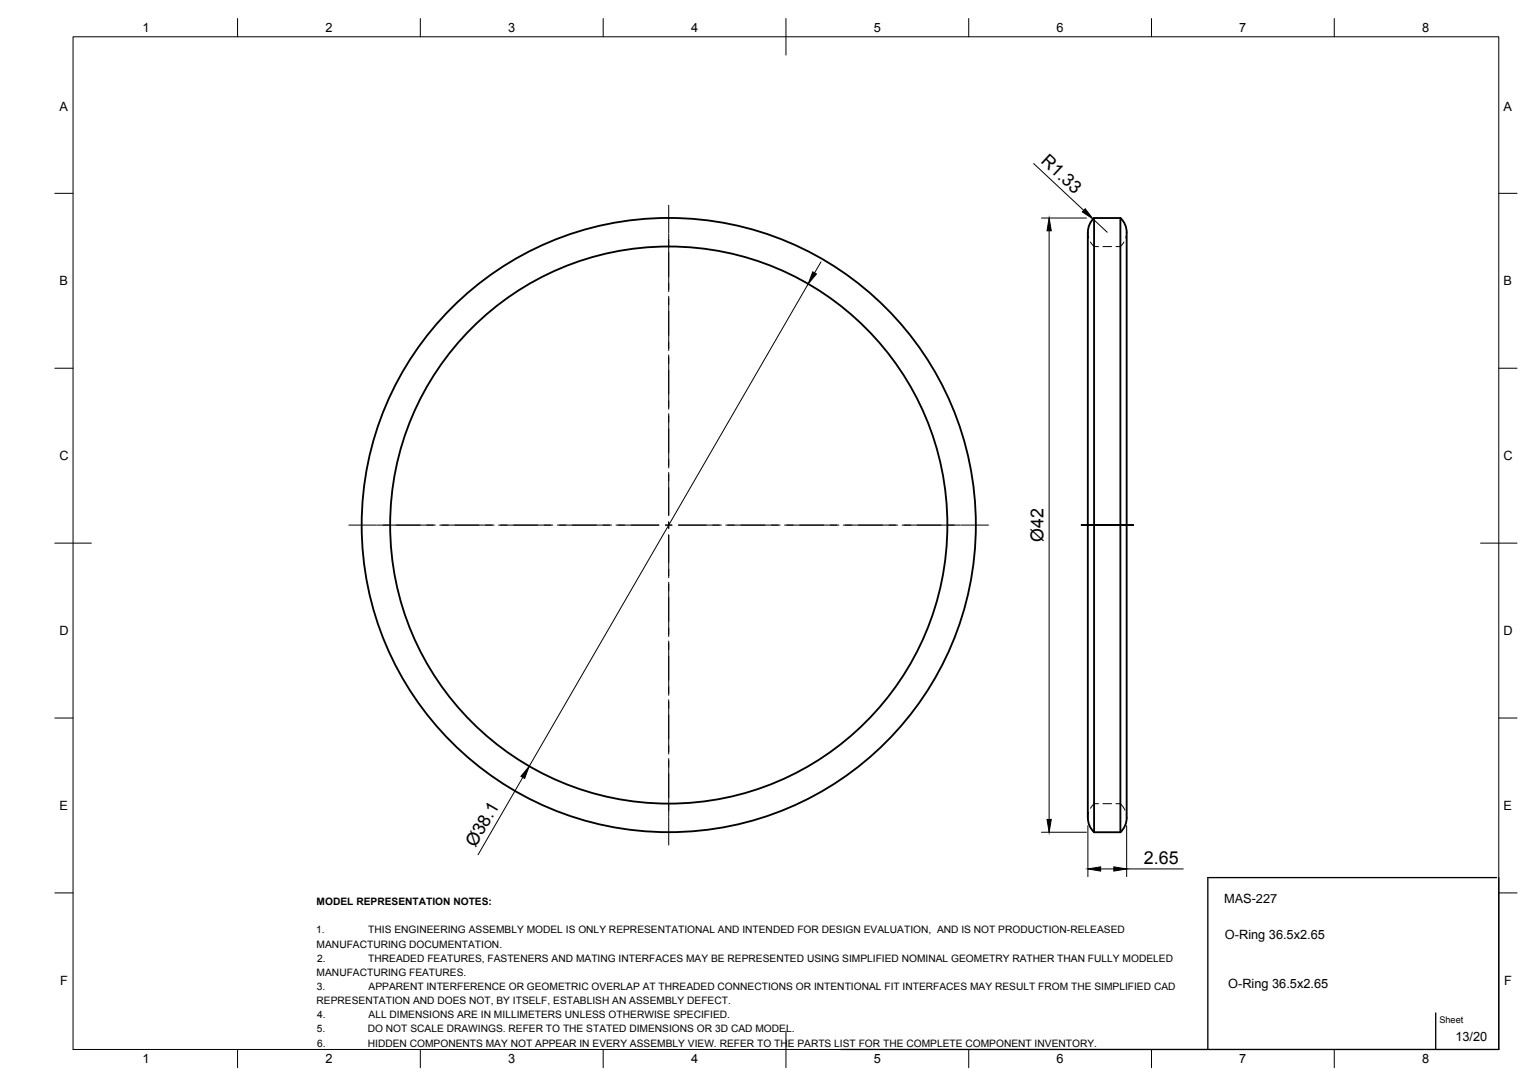
ISO-10303-21;
HEADER;
FILE_DESCRIPTION (('STEP AP214'),
    '1' );
FILE_NAME ( 'O-Ring 36.5x2.65.step', '2026-10-06T08:24:41', ( '' ), ( '' ), 'STEP AP214', 'Unspecified', '' );
FILE_SCHEMA (( 'AUTOMOTIVE_DESIGN' ));
ENDSEC;
DATA;
#54=DIRECTION ( 'NONE',  ( 1.000000000000000000, 0.000000000000000000, 0.000000000000000000 ) ) ;
#154=ADVANCED_FACE ( 'NONE', ( #2979 ), #26440, .T. ) ;
#275=ORIENTED_EDGE ( 'NONE', *, *, #12081, .F. ) ;
#358=DIRECTION ( 'NONE',  ( 0.000000000000000000, 0.000000000000000000, -1.000000000000000000 ) ) ;
#727=AXIS2_PLACEMENT_3D ( 'NONE', #14437, #3821, #3372 ) ;
#893=DIRECTION ( 'NONE',  ( 0.000000000000000000, 1.000000000000000000, 0.000000000000000000 ) ) ;
#953=DIRECTION ( 'NONE',  ( 1.000000000000000000, 0.000000000000000000, 0.000000000000000000 ) ) ;
#1494=CARTESIAN_POINT ( 'NONE',  ( -0.03532354024591893848, -0.07677165354330710290, 0.000000000000000000 ) ) ;
#1499=ORIENTED_EDGE ( 'NONE', *, *, #6385, .T. ) ;
#1533=PRODUCT_DEFINITION ( 'UNKNOWN', '', #2104, #3431 ) ;
#1669=ORIENTED_EDGE ( 'NONE', *, *, #3115, .T. ) ;
#1764=DIRECTION ( 'NONE',  ( 0.000000000000000000, 1.000000000000000000, 0.000000000000000000 ) ) ;
#1788=EDGE_CURVE ( 'NONE', #6256, #18898, #12424, .T. ) ;
#1859=ORIENTED_EDGE ( 'NONE', *, *, #22214, .F. ) ;
#1926=DIRECTION ( 'NONE',  ( 1.000000000000000000, 0.000000000000000000, 0.000000000000000000 ) ) ;
#2043=EDGE_CURVE ( 'NONE', #17434, #11924, #21465, .T. ) ;
#2104=PRODUCT_DEFINITION_FORMATION_WITH_SPECIFIED_SOURCE ( 'ANY', '', #22884, .NOT_KNOWN. ) ;
#2296=CARTESIAN_POINT ( 'NONE',  ( -9.069736220472442904E-16, -0.8267716535433071723, 0.000000000000000000 ) ) ;
#2375=EDGE_LOOP ( 'NONE', ( #25682, #7320, #24025, #12399, #13275, #4753 ) ) ;
#2557=ORIENTED_EDGE ( 'NONE', *, *, #12567, .F. ) ;
#2568=FACE_OUTER_BOUND ( 'NONE', #25010, .T. ) ;
#2659=ORIENTED_EDGE ( 'NONE', *, *, #23278, .F. ) ;
#2715=AXIS2_PLACEMENT_3D ( 'NONE', #11396, #22136, #24804 ) ;
#2813=AXIS2_PLACEMENT_3D ( 'NONE', #9732, #3355, #3801 ) ;
#2979=FACE_OUTER_BOUND ( 'NONE', #26175, .T. ) ;
#3059=( CONVERSION_BASED_UNIT ( 'INCH', #5779 ) LENGTH_UNIT ( ) NAMED_UNIT ( #6927 ) ) ;
#3098=EDGE_CURVE ( 'NONE', #18478, #18898, #7298, .T. ) ;
#3105=APPLICATION_CONTEXT ( 'automotive_design' ) ;
#3115=EDGE_CURVE ( 'NONE', #27881, #10521, #9696, .T. ) ;
#3269=DIRECTION ( 'NONE',  ( 0.000000000000000000, 1.000000000000000000, 0.000000000000000000 ) ) ;
#3355=DIRECTION ( 'NONE',  ( 1.000000000000000000, 0.000000000000000000, 0.000000000000000000 ) ) ;
#3372=DIRECTION ( 'NONE',  ( 1.000000000000000000, 0.000000000000000000, 0.000000000000000000 ) ) ;
#3431=PRODUCT_DEFINITION_CONTEXT ( 'detailed design', #3105, 'design' ) ;
#3439=DIRECTION ( 'NONE',  ( 1.000000000000000000, 0.000000000000000000, 0.000000000000000000 ) ) ;
#3497=VECTOR ( 'NONE', #20294, 39.37007874015748143 ) ;
#3512=AXIS2_PLACEMENT_3D ( 'NONE', #10785, #15718, #19545 ) ;
#3517=ORIENTED_EDGE ( 'NONE', *, *, #3621, .T. ) ;
#3592=ADVANCED_FACE ( 'NONE', ( #2568 ), #20689, .T. ) ;
#3621=EDGE_CURVE ( 'NONE', #16090, #10521, #23858, .T. ) ;
#3665=DIRECTION ( 'NONE',  ( 0.000000000000000000, 0.000000000000000000, 1.000000000000000000 ) ) ;
#3718=ORIENTED_EDGE ( 'NONE', *, *, #6749, .F. ) ;
#3738=CIRCLE ( 'NONE', #17721, 0.7500000000000001110 ) ;
#3801=DIRECTION ( 'NONE',  ( 0.000000000000000000, 1.000000000000000000, 0.000000000000000000 ) ) ;
#3821=DIRECTION ( 'NONE',  ( -1.147443000000000016E-15, -1.000000000000000000, -0.000000000000000000 ) ) ;
#4013=DIRECTION ( 'NONE',  ( 1.147443000000000016E-15, 1.000000000000000000, -1.224646799147353207E-16 ) ) ;
#4081=ORIENTED_EDGE ( 'NONE', *, *, #2043, .T. ) ;
#4143=COLOUR_RGB ( '', 0.31764706, 0.68627451, 0.89019608) ;
#4379=CIRCLE ( 'NONE', #4458, 0.7500000000000001110 ) ;
#4413=AXIS2_PLACEMENT_3D ( 'NONE', #15060, #6843, #7242 ) ;
#4458=AXIS2_PLACEMENT_3D ( 'NONE', #13653, #953, #22137 ) ;
#4753=ORIENTED_EDGE ( 'NONE', *, *, #15365, .F. ) ;
#5004=AXIS2_PLACEMENT_3D ( 'NONE', #6179, #23951, #19289 ) ;
#5229=CARTESIAN_POINT ( 'NONE',  ( 0.000000000000000000, 0.000000000000000000, 0.000000000000000000 ) ) ;
#5350=CIRCLE ( 'NONE', #9865, 0.8267716535433071723 ) ;
#5380=CIRCLE ( 'NONE', #23912, 0.7500000000000001110 ) ;
#5383=CARTESIAN_POINT ( 'NONE',  ( -9.069736220472440932E-16, -0.8267716535433070613, 0.7883858267716535861 ) ) ;
#5415=SHAPE_REPRESENTATION ( 'O-Ring 36.5x2.65', ( #11588 ), #12073 ) ;
#5431=CARTESIAN_POINT ( 'NONE',  ( -0.03532354024591901481, -0.8267716535433070613, 0.8267716535433070613 ) ) ;
#5548=TOROIDAL_SURFACE ( 'NONE', #20874, 0.7883858267716535861, 0.05216535433070866590 ) ;
#5658=AXIS2_PLACEMENT_3D ( 'NONE', #16841, #14751, #17254 ) ;
#5779=LENGTH_MEASURE_WITH_UNIT ( LENGTH_MEASURE( 0.02539999999999999897 ), #11694 ) ;
#5900=CARTESIAN_POINT ( 'NONE',  ( 0.03532354024591720376, -0.07677165354330710290, 0.000000000000000000 ) ) ;
#5969=DIRECTION ( 'NONE',  ( 1.000000000000000000, 0.000000000000000000, 0.000000000000000000 ) ) ;
#6179=CARTESIAN_POINT ( 'NONE',  ( 0.03532354024591720376, -0.8267716535433071723, 0.000000000000000000 ) ) ;
#6256=VERTEX_POINT ( 'NONE', #16209 ) ;
#6276=VERTEX_POINT ( 'NONE', #5900 ) ;
#6323=VECTOR ( 'NONE', #1926, 39.37007874015748143 ) ;
#6347=AXIS2_PLACEMENT_3D ( 'NONE', #26823, #11849, #7473 ) ;
#6385=EDGE_CURVE ( 'NONE', #17999, #18223, #25936, .T. ) ;
#6400=EDGE_LOOP ( 'NONE', ( #14006, #9282, #3718, #18640, #19761, #26637 ) ) ;
#6472=EDGE_LOOP ( 'NONE', ( #24744, #21279, #20965, #19101, #24711, #8476 ) ) ;
#6507=ORIENTED_EDGE ( 'NONE', *, *, #8834, .F. ) ;
#6607=CIRCLE ( 'NONE', #727, 0.05216535433070866590 ) ;
#6629=ADVANCED_FACE ( 'NONE', ( #27518 ), #24064, .F. ) ;
#6697=DIRECTION ( 'NONE',  ( 1.000000000000000000, 0.000000000000000000, 0.000000000000000000 ) ) ;
#6749=EDGE_CURVE ( 'NONE', #11924, #14095, #11728, .T. ) ;
#6843=DIRECTION ( 'NONE',  ( 1.000000000000000000, 0.000000000000000000, 0.000000000000000000 ) ) ;
#6927=DIMENSIONAL_EXPONENTS ( 1.000000000000000000, 0.000000000000000000, 0.000000000000000000, 0.000000000000000000, 0.000000000000000000, 0.000000000000000000, 0.000000000000000000 ) ;
#6933=SURFACE_SIDE_STYLE ('',( #26000 ) ) ;
#7013=AXIS2_PLACEMENT_3D ( 'NONE', #26658, #20166, #26383 ) ;
#7106=CARTESIAN_POINT ( 'NONE',  ( -9.506830708661417994E-16, -0.8267716535433071723, 0.000000000000000000 ) ) ;
#7112=CARTESIAN_POINT ( 'NONE',  ( 0.03532354024591712049, -0.8267716535433071723, 0.000000000000000000 ) ) ;
#7199=CIRCLE ( 'NONE', #9438, 0.7500000000000001110 ) ;
#7242=DIRECTION ( 'NONE',  ( 0.000000000000000000, 1.000000000000000000, 0.000000000000000000 ) ) ;
#7259=ADVANCED_FACE ( 'NONE', ( #13509 ), #7434, .F. ) ;
#7265=CARTESIAN_POINT ( 'NONE',  ( -9.069736220472442904E-16, -0.8267716535433071723, 0.000000000000000000 ) ) ;
#7298=LINE ( 'NONE', #9261, #3497 ) ;
#7320=ORIENTED_EDGE ( 'NONE', *, *, #18108, .T. ) ;
#7427=DIRECTION ( 'NONE',  ( 0.000000000000000000, 1.000000000000000000, 0.000000000000000000 ) ) ;
#7434=CYLINDRICAL_SURFACE ( 'NONE', #2715, 0.7500000000000001110 ) ;
#7473=DIRECTION ( 'NONE',  ( 0.000000000000000000, 1.000000000000000000, 0.000000000000000000 ) ) ;
#7497=AXIS2_PLACEMENT_3D ( 'NONE', #22749, #18351, #12293 ) ;
#7529=DIRECTION ( 'NONE',  ( 1.000000000000000000, 0.000000000000000000, 0.000000000000000000 ) ) ;
#7625=CYLINDRICAL_SURFACE ( 'NONE', #2813, 0.8267716535433071723 ) ;
#7667=ORIENTED_EDGE ( 'NONE', *, *, #20733, .T. ) ;
#7694=ORIENTED_EDGE ( 'NONE', *, *, #23278, .T. ) ;
#7752=EDGE_LOOP ( 'NONE', ( #7667, #22292, #1669, #20527, #1859, #13973 ) ) ;
#7757=EDGE_CURVE ( 'NONE', #23920, #6276, #9061, .T. ) ;
#7770=PRODUCT_DEFINITION_SHAPE ( 'NONE', 'NONE',  #1533 ) ;
#7923=DIRECTION ( 'NONE',  ( 1.000000000000000000, 0.000000000000000000, 0.000000000000000000 ) ) ;
#7957=VERTEX_POINT ( 'NONE', #5431 ) ;
#7970=ORIENTED_EDGE ( 'NONE', *, *, #2043, .F. ) ;
#8012=CARTESIAN_POINT ( 'NONE',  ( 0.03532354024591720376, -1.576771653543307172, 9.184850993605150903E-17 ) ) ;
#8080=CARTESIAN_POINT ( 'NONE',  ( -0.03532354024591893848, -0.8267716535433071723, -0.7500000000000001110 ) ) ;
#8084=CARTESIAN_POINT ( 'NONE',  ( 0.03532354024591712049, -0.8267716535433071723, 0.000000000000000000 ) ) ;
#8218=DIRECTION ( 'NONE',  ( 1.000000000000000000, 0.000000000000000000, 0.000000000000000000 ) ) ;
#8410=DIRECTION ( 'NONE',  ( 1.000000000000000000, 0.000000000000000000, 0.000000000000000000 ) ) ;
#8476=ORIENTED_EDGE ( 'NONE', *, *, #1788, .T. ) ;
#8487=( CONVERSION_BASED_UNIT ( 'INCH', #10883 ) LENGTH_UNIT ( ) NAMED_UNIT ( #22953 ) ) ;
#8506=EDGE_CURVE ( 'NONE', #14095, #7957, #15004, .T. ) ;
#8613=DIRECTION ( 'NONE',  ( 1.000000000000000000, 0.000000000000000000, 0.000000000000000000 ) ) ;
#8620=DIRECTION ( 'NONE',  ( 0.000000000000000000, 1.000000000000000000, 0.000000000000000000 ) ) ;
#8834=EDGE_CURVE ( 'NONE', #11924, #6276, #27573, .T. ) ;
#8969=FACE_OUTER_BOUND ( 'NONE', #16226, .T. ) ;
#9030=FILL_AREA_STYLE_COLOUR ( '', #4143 ) ;
#9061=CIRCLE ( 'NONE', #5004, 0.7500000000000001110 ) ;
#9258=ADVANCED_FACE ( 'NONE', ( #16380 ), #7625, .T. ) ;
#9261=CARTESIAN_POINT ( 'NONE',  ( -9.506830708661417994E-16, 0.000000000000000000, 0.000000000000000000 ) ) ;
#9282=ORIENTED_EDGE ( 'NONE', *, *, #18108, .F. ) ;
#9337=DIRECTION ( 'NONE',  ( 1.000000000000000000, 0.000000000000000000, 0.000000000000000000 ) ) ;
#9392=DIRECTION ( 'NONE',  ( 1.000000000000000000, 0.000000000000000000, 0.000000000000000000 ) ) ;
#9438=AXIS2_PLACEMENT_3D ( 'NONE', #21199, #8613, #27031 ) ;
#9531=VECTOR ( 'NONE', #8218, 39.37007874015748143 ) ;
#9601=DIRECTION ( 'NONE',  ( 1.147443000000000016E-15, 1.000000000000000000, -1.224646799147353207E-16 ) ) ;
#9630=DIRECTION ( 'NONE',  ( 0.000000000000000000, 1.000000000000000000, 0.000000000000000000 ) ) ;
#9696=LINE ( 'NONE', #18296, #11621 ) ;
#9732=CARTESIAN_POINT ( 'NONE',  ( -9.506830708661417994E-16, -0.8267716535433071723, 0.000000000000000000 ) ) ;
#9750=CARTESIAN_POINT ( 'NONE',  ( -0.03532354024591901481, -1.653543307086614345, 1.012503259137575512E-16 ) ) ;
#9859=( NAMED_UNIT ( * ) SI_UNIT ( $, .STERADIAN. ) SOLID_ANGLE_UNIT ( ) ) ;
#9865=AXIS2_PLACEMENT_3D ( 'NONE', #19355, #54, #8620 ) ;
#10041=CARTESIAN_POINT ( 'NONE',  ( -8.632637795275590524E-16, -0.07677165354330710290, 0.000000000000000000 ) ) ;
#10188=CIRCLE ( 'NONE', #21950, 0.05216535433070866590 ) ;
#10458=AXIS2_PLACEMENT_3D ( 'NONE', #27460, #4013, #20958 ) ;
#10521=VERTEX_POINT ( 'NONE', #17065 ) ;
#10785=CARTESIAN_POINT ( 'NONE',  ( 0.03532354024591712049, -0.8267716535433071723, 0.000000000000000000 ) ) ;
#10857=AXIS2_PLACEMENT_3D ( 'NONE', #15408, #16853, #18661 ) ;
#10883=LENGTH_MEASURE_WITH_UNIT ( LENGTH_MEASURE( 0.02539999999999999897 ), #19498 ) ;
#11131=ORIENTED_EDGE ( 'NONE', *, *, #11690, .F. ) ;
#11208=AXIS2_PLACEMENT_3D ( 'NONE', #8084, #5969, #18942 ) ;
#11396=CARTESIAN_POINT ( 'NONE',  ( -8.632637795275590524E-16, -0.8267716535433071723, 0.000000000000000000 ) ) ;
#11588=AXIS2_PLACEMENT_3D ( 'NONE', #5229, #3665, #7923 ) ;
#11621=VECTOR ( 'NONE', #22138, 39.37007874015748143 ) ;
#11690=EDGE_CURVE ( 'NONE', #18223, #23920, #3738, .T. ) ;
#11694=( LENGTH_UNIT ( ) NAMED_UNIT ( * ) SI_UNIT ( $, .METRE. ) ) ;
#11728=CIRCLE ( 'NONE', #6347, 0.7500000000000001110 ) ;
#11849=DIRECTION ( 'NONE',  ( 1.000000000000000000, 0.000000000000000000, 0.000000000000000000 ) ) ;
#11924=VERTEX_POINT ( 'NONE', #1494 ) ;
#11936=CIRCLE ( 'NONE', #18673, 0.8267716535433071723 ) ;
#11990=VERTEX_POINT ( 'NONE', #22499 ) ;
#12073=( GEOMETRIC_REPRESENTATION_CONTEXT ( 3 ) GLOBAL_UNCERTAINTY_ASSIGNED_CONTEXT ( ( #18691 ) ) GLOBAL_UNIT_ASSIGNED_CONTEXT ( ( #3059, #16228, #9859 ) ) REPRESENTATION_CONTEXT ( 'NONE', 'WORKASPACE' ) ) ;
#12081=EDGE_CURVE ( 'NONE', #17434, #14806, #21229, .T. ) ;
#12293=DIRECTION ( 'NONE',  ( 0.000000000000000000, 0.000000000000000000, -1.000000000000000000 ) ) ;
#12381=CARTESIAN_POINT ( 'NONE',  ( -8.632637795275590524E-16, -1.576771653543307172, 9.184850993605150903E-17 ) ) ;
#12399=ORIENTED_EDGE ( 'NONE', *, *, #12081, .T. ) ;
#12424=CIRCLE ( 'NONE', #19193, 0.8267716535433071723 ) ;
#12567=EDGE_CURVE ( 'NONE', #11990, #18223, #21732, .T. ) ;
#12719=FILL_AREA_STYLE ('',( #9030 ) ) ;
#12811=ORIENTED_EDGE ( 'NONE', *, *, #22158, .T. ) ;
#13232=ORIENTED_EDGE ( 'NONE', *, *, #6749, .T. ) ;
#13259=ADVANCED_FACE ( 'NONE', ( #8969 ), #5548, .T. ) ;
#13275=ORIENTED_EDGE ( 'NONE', *, *, #19557, .F. ) ;
#13364=ORIENTED_EDGE ( 'NONE', *, *, #22350, .F. ) ;
#13390=DIRECTION ( 'NONE',  ( 0.000000000000000000, 1.000000000000000000, 0.000000000000000000 ) ) ;
#13444=DIRECTION ( 'NONE',  ( 1.000000000000000000, -1.147443000000000016E-15, 0.000000000000000000 ) ) ;
#13509=FACE_OUTER_BOUND ( 'NONE', #6400, .T. ) ;
#13515=CARTESIAN_POINT ( 'NONE',  ( 0.03532354024591720376, -0.8267716535433071723, -0.7500000000000001110 ) ) ;
#13653=CARTESIAN_POINT ( 'NONE',  ( -0.03532354024591893848, -0.8267716535433071723, 0.000000000000000000 ) ) ;
#13973=ORIENTED_EDGE ( 'NONE', *, *, #3098, .F. ) ;
#14006=ORIENTED_EDGE ( 'NONE', *, *, #6385, .F. ) ;
#14057=STYLED_ITEM ( 'NONE', ( #21627 ), #21602 ) ;
#14095=VERTEX_POINT ( 'NONE', #17627 ) ;
#14303=ORIENTED_EDGE ( 'NONE', *, *, #3098, .T. ) ;
#14351=CARTESIAN_POINT ( 'NONE',  ( 0.03532354024591720376, -0.8267716535433071723, 0.000000000000000000 ) ) ;
#14437=CARTESIAN_POINT ( 'NONE',  ( -9.069736220472442904E-16, -0.8267716535433071723, -0.7883858267716535861 ) ) ;
#14453=ORIENTED_EDGE ( 'NONE', *, *, #7757, .T. ) ;
#14655=CARTESIAN_POINT ( 'NONE',  ( -0.03532354024591901481, -0.8267716535433071723, 0.000000000000000000 ) ) ;
#14695=SHAPE_REPRESENTATION_RELATIONSHIP ( 'NONE' , 'NONE' ,  #5415, #17421 ) ;
#14751=DIRECTION ( 'NONE',  ( 1.000000000000000000, -1.147443000000000016E-15, 0.000000000000000000 ) ) ;
#14806=VERTEX_POINT ( 'NONE', #15024 ) ;
#14979=CARTESIAN_POINT ( 'NONE',  ( -0.03532354024591893848, -1.576771653543307172, 9.184850993605150903E-17 ) ) ;
#15004=CIRCLE ( 'NONE', #10458, 0.05216535433070866590 ) ;
#15024=CARTESIAN_POINT ( 'NONE',  ( -0.03532354024591901481, -0.8267716535433071723, -0.8267716535433070613 ) ) ;
#15060=CARTESIAN_POINT ( 'NONE',  ( -0.03532354024591901481, -0.8267716535433071723, 0.000000000000000000 ) ) ;
#15184=TOROIDAL_SURFACE ( 'NONE', #7497, 0.7883858267716535861, 0.05216535433070866590 ) ;
#15256=AXIS2_PLACEMENT_3D ( 'NONE', #7112, #7529, #3269 ) ;
#15365=EDGE_CURVE ( 'NONE', #7957, #27881, #11936, .T. ) ;
#15408=CARTESIAN_POINT ( 'NONE',  ( -9.069736220472442904E-16, -0.8267716535433071723, -0.7883858267716535861 ) ) ;
#15522=AXIS2_PLACEMENT_3D ( 'NONE', #7106, #9337, #893 ) ;
#15555=( NAMED_UNIT ( * ) SI_UNIT ( $, .STERADIAN. ) SOLID_ANGLE_UNIT ( ) ) ;
#15607=AXIS2_PLACEMENT_3D ( 'NONE', #14655, #8410, #1764 ) ;
#15718=DIRECTION ( 'NONE',  ( 1.000000000000000000, 0.000000000000000000, 0.000000000000000000 ) ) ;
#15731=AXIS2_PLACEMENT_3D ( 'NONE', #2296, #13444, #358 ) ;
#15932=PRODUCT_CONTEXT ( 'NONE', #19177, 'mechanical' ) ;
#16062=CIRCLE ( 'NONE', #15607, 0.8267716535433071723 ) ;
#16090=VERTEX_POINT ( 'NONE', #27314 ) ;
#16124=DIRECTION ( 'NONE',  ( -1.000000000000000000, 0.000000000000000000, 0.000000000000000000 ) ) ;
#16209=CARTESIAN_POINT ( 'NONE',  ( 0.03532354024591712049, -0.8267716535433071723, -0.8267716535433071723 ) ) ;
#16226=EDGE_LOOP ( 'NONE', ( #24644, #3517, #7694, #23020, #11131, #2557 ) ) ;
#16228=( NAMED_UNIT ( * ) PLANE_ANGLE_UNIT ( ) SI_UNIT ( $, .RADIAN. ) ) ;
#16380=FACE_OUTER_BOUND ( 'NONE', #7752, .T. ) ;
#16405=CLOSED_SHELL ( 'NONE', ( #25676, #6629, #3592, #9258, #154, #26630, #7259, #13259 ) ) ;
#16567=ORIENTED_EDGE ( 'NONE', *, *, #11690, .T. ) ;
#16579=CIRCLE ( 'NONE', #4413, 0.8267716535433071723 ) ;
#16841=CARTESIAN_POINT ( 'NONE',  ( -9.069736220472442904E-16, -0.8267716535433071723, 0.000000000000000000 ) ) ;
#16853=DIRECTION ( 'NONE',  ( -1.147443000000000016E-15, -1.000000000000000000, -0.000000000000000000 ) ) ;
#17065=CARTESIAN_POINT ( 'NONE',  ( 0.03532354024591712049, -1.653543307086614345, 1.012503259137575512E-16 ) ) ;
#17254=DIRECTION ( 'NONE',  ( 0.000000000000000000, 0.000000000000000000, -1.000000000000000000 ) ) ;
#17421=ADVANCED_BREP_SHAPE_REPRESENTATION ( 'O-Ring 36.5x2.65', ( #21602, #11588 ), #12073 ) ;
#17434=VERTEX_POINT ( 'NONE', #8080 ) ;
#17627=CARTESIAN_POINT ( 'NONE',  ( -0.03532354024591893848, -0.8267716535433070613, 0.7500000000000001110 ) ) ;
#17631=CARTESIAN_POINT ( 'NONE',  ( -0.03532354024591901481, -0.8267716535433071723, 0.000000000000000000 ) ) ;
#17690=DIRECTION ( 'NONE',  ( 0.000000000000000000, 1.000000000000000000, 0.000000000000000000 ) ) ;
#17721=AXIS2_PLACEMENT_3D ( 'NONE', #24936, #9392, #7427 ) ;
#17999=VERTEX_POINT ( 'NONE', #14979 ) ;
#18108=EDGE_CURVE ( 'NONE', #14095, #17999, #4379, .T. ) ;
#18171=CARTESIAN_POINT ( 'NONE',  ( 0.03532354024591720376, -0.8267716535433071723, 0.000000000000000000 ) ) ;
#18223=VERTEX_POINT ( 'NONE', #8012 ) ;
#18235=DIRECTION ( 'NONE',  ( 1.000000000000000000, 0.000000000000000000, 0.000000000000000000 ) ) ;
#18296=CARTESIAN_POINT ( 'NONE',  ( -9.506830708661417994E-16, -1.653543307086614345, 1.012503259137575512E-16 ) ) ;
#18351=DIRECTION ( 'NONE',  ( 1.000000000000000000, -1.147443000000000016E-15, 0.000000000000000000 ) ) ;
#18460=DIRECTION ( 'NONE',  ( 0.000000000000000000, 1.000000000000000000, 0.000000000000000000 ) ) ;
#18478=VERTEX_POINT ( 'NONE', #27783 ) ;
#18622=UNCERTAINTY_MEASURE_WITH_UNIT (LENGTH_MEASURE( 1.000000000000000082E-05 ), #8487, 'distance_accuracy_value', 'NONE') ;
#18640=ORIENTED_EDGE ( 'NONE', *, *, #8834, .T. ) ;
#18661=DIRECTION ( 'NONE',  ( 1.000000000000000000, 0.000000000000000000, 0.000000000000000000 ) ) ;
#18673=AXIS2_PLACEMENT_3D ( 'NONE', #17631, #22018, #13390 ) ;
#18691=UNCERTAINTY_MEASURE_WITH_UNIT (LENGTH_MEASURE( 1.000000000000000082E-05 ), #3059, 'distance_accuracy_value', 'NONE') ;
#18711=EDGE_CURVE ( 'NONE', #6276, #11990, #5380, .T. ) ;
#18898=VERTEX_POINT ( 'NONE', #22978 ) ;
#18942=DIRECTION ( 'NONE',  ( 0.000000000000000000, 1.000000000000000000, 0.000000000000000000 ) ) ;
#19005=ORIENTED_EDGE ( 'NONE', *, *, #8506, .T. ) ;
#19101=ORIENTED_EDGE ( 'NONE', *, *, #7757, .F. ) ;
#19177=APPLICATION_CONTEXT ( 'automotive_design' ) ;
#19193=AXIS2_PLACEMENT_3D ( 'NONE', #24750, #18235, #9630 ) ;
#19289=DIRECTION ( 'NONE',  ( 0.000000000000000000, 1.000000000000000000, 0.000000000000000000 ) ) ;
#19355=CARTESIAN_POINT ( 'NONE',  ( -0.03532354024591901481, -0.8267716535433071723, 0.000000000000000000 ) ) ;
#19498=( LENGTH_UNIT ( ) NAMED_UNIT ( * ) SI_UNIT ( $, .METRE. ) ) ;
#19545=DIRECTION ( 'NONE',  ( 0.000000000000000000, 1.000000000000000000, 0.000000000000000000 ) ) ;
#19557=EDGE_CURVE ( 'NONE', #27881, #14806, #16062, .T. ) ;
#19761=ORIENTED_EDGE ( 'NONE', *, *, #18711, .T. ) ;
#20044=ORIENTED_EDGE ( 'NONE', *, *, #20733, .F. ) ;
#20166=DIRECTION ( 'NONE',  ( 1.000000000000000000, 0.000000000000000000, 0.000000000000000000 ) ) ;
#20294=DIRECTION ( 'NONE',  ( 1.000000000000000000, 0.000000000000000000, 0.000000000000000000 ) ) ;
#20457=ORIENTED_EDGE ( 'NONE', *, *, #22158, .F. ) ;
#20493=FACE_OUTER_BOUND ( 'NONE', #2375, .T. ) ;
#20527=ORIENTED_EDGE ( 'NONE', *, *, #3621, .F. ) ;
#20530=TOROIDAL_SURFACE ( 'NONE', #5658, 0.7883858267716535861, 0.05216535433070866590 ) ;
#20689=TOROIDAL_SURFACE ( 'NONE', #15731, 0.7883858267716535861, 0.05216535433070866590 ) ;
#20733=EDGE_CURVE ( 'NONE', #18478, #7957, #5350, .T. ) ;
#20874=AXIS2_PLACEMENT_3D ( 'NONE', #7265, #24092, #24361 ) ;
#20958=DIRECTION ( 'NONE',  ( -1.000000000000000000, 0.000000000000000000, 0.000000000000000000 ) ) ;
#20965=ORIENTED_EDGE ( 'NONE', *, *, #18711, .F. ) ;
#21173=ORIENTED_EDGE ( 'NONE', *, *, #1788, .F. ) ;
#21199=CARTESIAN_POINT ( 'NONE',  ( -0.03532354024591893848, -0.8267716535433071723, 0.000000000000000000 ) ) ;
#21229=CIRCLE ( 'NONE', #10857, 0.05216535433070866590 ) ;
#21279=ORIENTED_EDGE ( 'NONE', *, *, #26777, .T. ) ;
#21290=( GEOMETRIC_REPRESENTATION_CONTEXT ( 3 ) GLOBAL_UNCERTAINTY_ASSIGNED_CONTEXT ( ( #18622 ) ) GLOBAL_UNIT_ASSIGNED_CONTEXT ( ( #8487, #21488, #15555 ) ) REPRESENTATION_CONTEXT ( 'NONE', 'WORKASPACE' ) ) ;
#21465=CIRCLE ( 'NONE', #7013, 0.7500000000000001110 ) ;
#21488=( NAMED_UNIT ( * ) PLANE_ANGLE_UNIT ( ) SI_UNIT ( $, .RADIAN. ) ) ;
#21533=CARTESIAN_POINT ( 'NONE',  ( -8.632637795275590524E-16, -0.8267716535433071723, 0.000000000000000000 ) ) ;
#21602=MANIFOLD_SOLID_BREP ( 'O-Ring 36.5x2.65', #16405 ) ;
#21627=PRESENTATION_STYLE_ASSIGNMENT (( #23894 ) ) ;
#21732=CIRCLE ( 'NONE', #24410, 0.7500000000000001110 ) ;
#21950=AXIS2_PLACEMENT_3D ( 'NONE', #5383, #9601, #16124 ) ;
#22018=DIRECTION ( 'NONE',  ( 1.000000000000000000, 0.000000000000000000, 0.000000000000000000 ) ) ;
#22136=DIRECTION ( 'NONE',  ( 1.000000000000000000, 0.000000000000000000, 0.000000000000000000 ) ) ;
#22137=DIRECTION ( 'NONE',  ( 0.000000000000000000, 1.000000000000000000, 0.000000000000000000 ) ) ;
#22138=DIRECTION ( 'NONE',  ( 1.000000000000000000, 0.000000000000000000, 0.000000000000000000 ) ) ;
#22158=EDGE_CURVE ( 'NONE', #14806, #18478, #16579, .T. ) ;
#22214=EDGE_CURVE ( 'NONE', #18898, #16090, #27417, .T. ) ;
#22292=ORIENTED_EDGE ( 'NONE', *, *, #15365, .T. ) ;
#22350=EDGE_CURVE ( 'NONE', #17999, #17434, #7199, .T. ) ;
#22499=CARTESIAN_POINT ( 'NONE',  ( 0.03532354024591720376, -0.8267716535433070613, 0.7500000000000001110 ) ) ;
#22749=CARTESIAN_POINT ( 'NONE',  ( -9.069736220472442904E-16, -0.8267716535433071723, 0.000000000000000000 ) ) ;
#22884=PRODUCT ( 'O-Ring 36.5x2.65', 'O-Ring 36.5x2.65', '', ( #15932 ) ) ;
#22953=DIMENSIONAL_EXPONENTS ( 1.000000000000000000, 0.000000000000000000, 0.000000000000000000, 0.000000000000000000, 0.000000000000000000, 0.000000000000000000, 0.000000000000000000 ) ;
#22978=CARTESIAN_POINT ( 'NONE',  ( 0.03532354024591712049, 0.000000000000000000, 0.000000000000000000 ) ) ;
#23020=ORIENTED_EDGE ( 'NONE', *, *, #26703, .T. ) ;
#23278=EDGE_CURVE ( 'NONE', #10521, #6256, #24439, .T. ) ;
#23431=SHAPE_DEFINITION_REPRESENTATION ( #7770, #5415 ) ;
#23479=AXIS2_PLACEMENT_3D ( 'NONE', #21533, #6697, #17690 ) ;
#23761=FACE_OUTER_BOUND ( 'NONE', #6472, .T. ) ;
#23858=CIRCLE ( 'NONE', #3512, 0.8267716535433071723 ) ;
#23894=SURFACE_STYLE_USAGE ( .BOTH. , #6933 ) ;
#23912=AXIS2_PLACEMENT_3D ( 'NONE', #18171, #24683, #18460 ) ;
#23920=VERTEX_POINT ( 'NONE', #13515 ) ;
#23951=DIRECTION ( 'NONE',  ( 1.000000000000000000, 0.000000000000000000, 0.000000000000000000 ) ) ;
#24000=ORIENTED_EDGE ( 'NONE', *, *, #3115, .F. ) ;
#24025=ORIENTED_EDGE ( 'NONE', *, *, #22350, .T. ) ;
#24064=CYLINDRICAL_SURFACE ( 'NONE', #23479, 0.7500000000000001110 ) ;
#24092=DIRECTION ( 'NONE',  ( 1.000000000000000000, -1.147443000000000016E-15, 0.000000000000000000 ) ) ;
#24361=DIRECTION ( 'NONE',  ( 0.000000000000000000, 0.000000000000000000, -1.000000000000000000 ) ) ;
#24410=AXIS2_PLACEMENT_3D ( 'NONE', #14351, #3439, #25637 ) ;
#24428=MECHANICAL_DESIGN_GEOMETRIC_PRESENTATION_REPRESENTATION('',(#14057),#21290);
#24439=CIRCLE ( 'NONE', #11208, 0.8267716535433071723 ) ;
#24644=ORIENTED_EDGE ( 'NONE', *, *, #26777, .F. ) ;
#24683=DIRECTION ( 'NONE',  ( 1.000000000000000000, 0.000000000000000000, 0.000000000000000000 ) ) ;
#24711=ORIENTED_EDGE ( 'NONE', *, *, #26703, .F. ) ;
#24744=ORIENTED_EDGE ( 'NONE', *, *, #22214, .T. ) ;
#24750=CARTESIAN_POINT ( 'NONE',  ( 0.03532354024591712049, -0.8267716535433071723, 0.000000000000000000 ) ) ;
#24804=DIRECTION ( 'NONE',  ( 0.000000000000000000, 1.000000000000000000, 0.000000000000000000 ) ) ;
#24936=CARTESIAN_POINT ( 'NONE',  ( 0.03532354024591720376, -0.8267716535433071723, 0.000000000000000000 ) ) ;
#25010=EDGE_LOOP ( 'NONE', ( #4081, #13232, #19005, #20044, #20457, #275 ) ) ;
#25197=ORIENTED_EDGE ( 'NONE', *, *, #19557, .T. ) ;
#25637=DIRECTION ( 'NONE',  ( 0.000000000000000000, 1.000000000000000000, 0.000000000000000000 ) ) ;
#25676=ADVANCED_FACE ( 'NONE', ( #23761 ), #20530, .T. ) ;
#25682=ORIENTED_EDGE ( 'NONE', *, *, #8506, .F. ) ;
#25835=EDGE_LOOP ( 'NONE', ( #13364, #1499, #16567, #14453, #6507, #7970 ) ) ;
#25936=LINE ( 'NONE', #12381, #6323 ) ;
#26000=SURFACE_STYLE_FILL_AREA ( #12719 ) ;
#26175=EDGE_LOOP ( 'NONE', ( #24000, #25197, #12811, #14303, #21173, #2659 ) ) ;
#26383=DIRECTION ( 'NONE',  ( 0.000000000000000000, 1.000000000000000000, 0.000000000000000000 ) ) ;
#26440=CYLINDRICAL_SURFACE ( 'NONE', #15522, 0.8267716535433071723 ) ;
#26630=ADVANCED_FACE ( 'NONE', ( #20493 ), #15184, .T. ) ;
#26637=ORIENTED_EDGE ( 'NONE', *, *, #12567, .T. ) ;
#26658=CARTESIAN_POINT ( 'NONE',  ( -0.03532354024591893848, -0.8267716535433071723, 0.000000000000000000 ) ) ;
#26703=EDGE_CURVE ( 'NONE', #6256, #23920, #6607, .T. ) ;
#26777=EDGE_CURVE ( 'NONE', #16090, #11990, #10188, .T. ) ;
#26823=CARTESIAN_POINT ( 'NONE',  ( -0.03532354024591893848, -0.8267716535433071723, 0.000000000000000000 ) ) ;
#27031=DIRECTION ( 'NONE',  ( 0.000000000000000000, 1.000000000000000000, 0.000000000000000000 ) ) ;
#27314=CARTESIAN_POINT ( 'NONE',  ( 0.03532354024591712049, -0.8267716535433070613, 0.8267716535433071723 ) ) ;
#27417=CIRCLE ( 'NONE', #15256, 0.8267716535433071723 ) ;
#27460=CARTESIAN_POINT ( 'NONE',  ( -9.069736220472440932E-16, -0.8267716535433070613, 0.7883858267716535861 ) ) ;
#27518=FACE_OUTER_BOUND ( 'NONE', #25835, .T. ) ;
#27573=LINE ( 'NONE', #10041, #9531 ) ;
#27783=CARTESIAN_POINT ( 'NONE',  ( -0.03532354024591901481, 0.000000000000000000, 0.000000000000000000 ) ) ;
#27881=VERTEX_POINT ( 'NONE', #9750 ) ;
ENDSEC;
END-ISO-10303-21;
